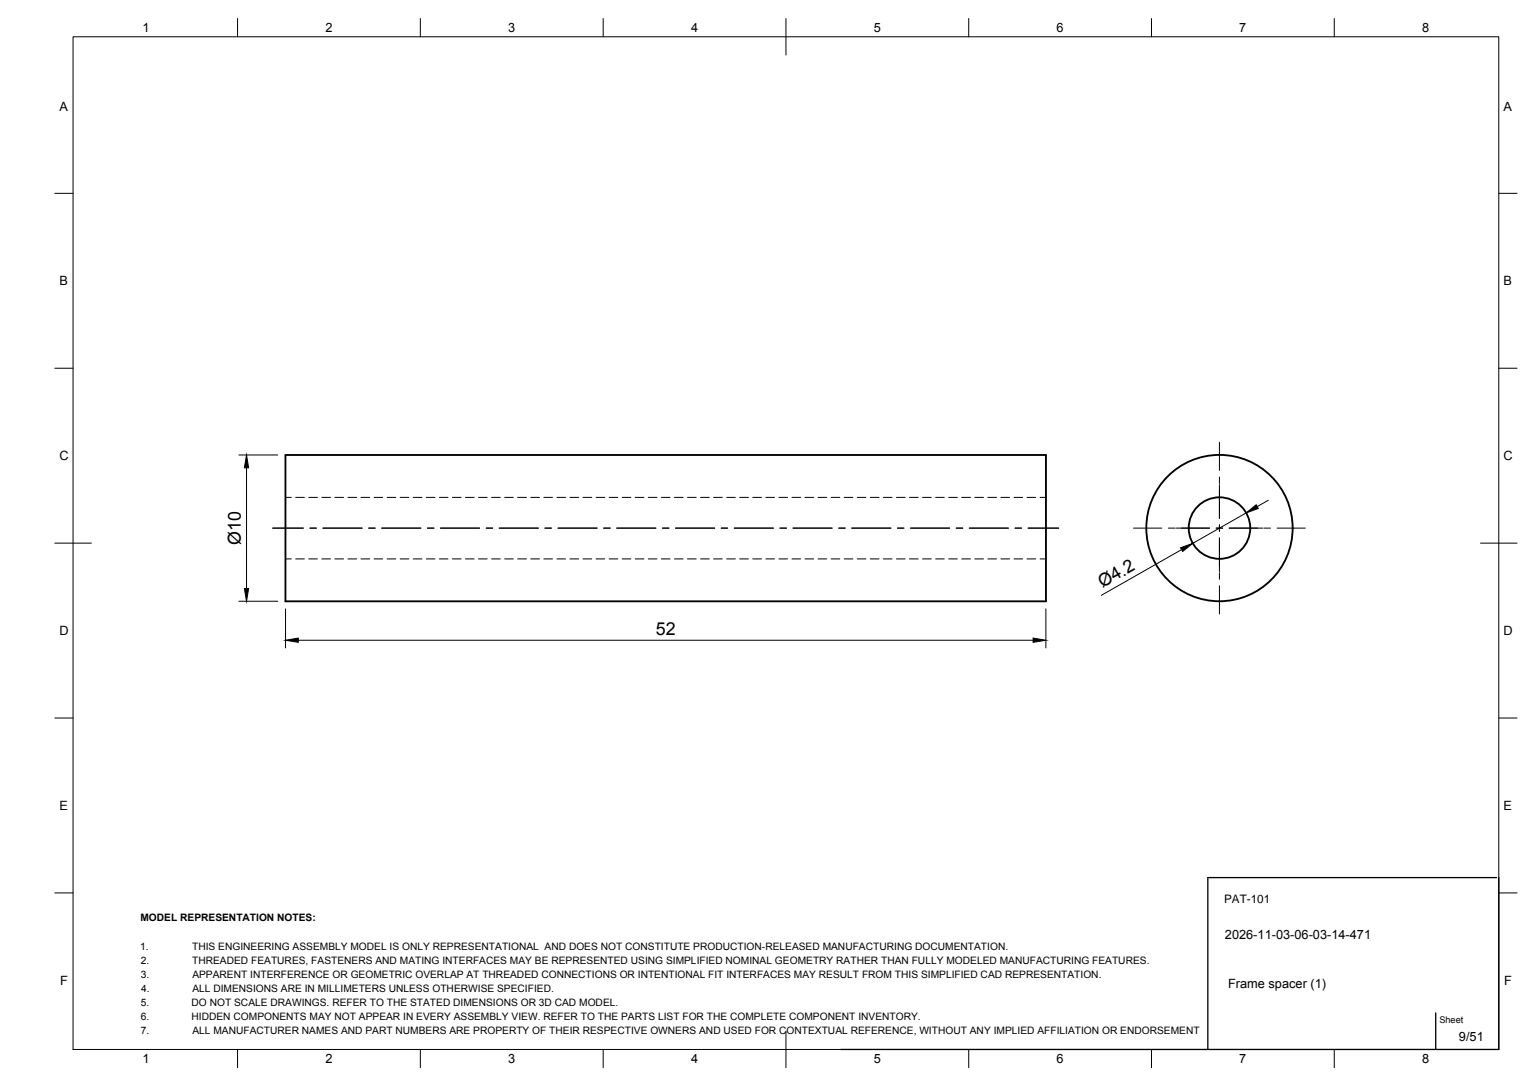
ISO-10303-21;
HEADER;
/* Generated by software containing ST-Developer
 * from STEP Tools, Inc. (www.steptools.com) 
 */

FILE_DESCRIPTION(
/* description */ ('Spur gear reduction stage 2-1 on bearing plates'),
/* implementation_level */ '2;1');

FILE_NAME(
/* name */ 'Frame spacer (1).step',
/* time_stamp */ '2026-10-28T03:22:07-07:00',
/* author */ (''),
/* organization */ (''),
/* preprocessor_version */ 'ST-DEVELOPER v20.2',
/* originating_system */ 'Autodesk Translation Framework v15.17.0.0',
/* authorisation */ '');

FILE_SCHEMA (('AUTOMOTIVE_DESIGN { 1 0 10303 214 3 1 1 }'));
ENDSEC;

DATA;
#10=MECHANICAL_DESIGN_GEOMETRIC_PRESENTATION_REPRESENTATION('',(#951),#53909);
#865=SHAPE_REPRESENTATION_RELATIONSHIP('SRR','None',#54092,#908);
#908=ADVANCED_BREP_SHAPE_REPRESENTATION('',(#1009),#53866);
#951=STYLED_ITEM('',(#54376),#1009);
#1009=MANIFOLD_SOLID_BREP('Body1',#11275);
#1134=FACE_BOUND('',#2310,.T.);
#1135=FACE_BOUND('',#2312,.T.);
#1274=PLANE('',#11993);
#1275=PLANE('',#11994);
#1585=FACE_OUTER_BOUND('',#2307,.T.);
#1586=FACE_OUTER_BOUND('',#2308,.T.);
#1587=FACE_OUTER_BOUND('',#2309,.T.);
#1588=FACE_OUTER_BOUND('',#2311,.T.);
#2307=EDGE_LOOP('',(#7700,#7701,#7702,#7703));
#2308=EDGE_LOOP('',(#7704,#7705,#7706,#7707));
#2309=EDGE_LOOP('',(#7708));
#2310=EDGE_LOOP('',(#7709));
#2311=EDGE_LOOP('',(#7710));
#2312=EDGE_LOOP('',(#7711));
#3059=LINE('',#16358,#3700);
#3060=LINE('',#16364,#3701);
#3700=VECTOR('',#13430,0.21);
#3701=VECTOR('',#13437,0.5);
#4351=CIRCLE('',#11988,0.21);
#4352=CIRCLE('',#11989,0.21);
#4353=CIRCLE('',#11991,0.5);
#4354=CIRCLE('',#11992,0.5);
#4900=VERTEX_POINT('',#16355);
#4901=VERTEX_POINT('',#16357);
#4902=VERTEX_POINT('',#16361);
#4903=VERTEX_POINT('',#16363);
#5992=EDGE_CURVE('',#4900,#4900,#4351,.T.);
#5993=EDGE_CURVE('',#4900,#4901,#3059,.T.);
#5994=EDGE_CURVE('',#4901,#4901,#4352,.T.);
#5995=EDGE_CURVE('',#4902,#4902,#4353,.T.);
#5996=EDGE_CURVE('',#4902,#4903,#3060,.T.);
#5997=EDGE_CURVE('',#4903,#4903,#4354,.T.);
#7700=ORIENTED_EDGE('',*,*,#5992,.F.);
#7701=ORIENTED_EDGE('',*,*,#5993,.T.);
#7702=ORIENTED_EDGE('',*,*,#5994,.T.);
#7703=ORIENTED_EDGE('',*,*,#5993,.F.);
#7704=ORIENTED_EDGE('',*,*,#5995,.F.);
#7705=ORIENTED_EDGE('',*,*,#5996,.T.);
#7706=ORIENTED_EDGE('',*,*,#5997,.T.);
#7707=ORIENTED_EDGE('',*,*,#5996,.F.);
#7708=ORIENTED_EDGE('',*,*,#5995,.T.);
#7709=ORIENTED_EDGE('',*,*,#5992,.T.);
#7710=ORIENTED_EDGE('',*,*,#5997,.F.);
#7711=ORIENTED_EDGE('',*,*,#5994,.F.);
#10466=CYLINDRICAL_SURFACE('',#11987,0.21);
#10467=CYLINDRICAL_SURFACE('',#11990,0.5);
#10705=ADVANCED_FACE('',(#1585),#10466,.F.);
#10706=ADVANCED_FACE('',(#1586),#10467,.T.);
#10707=ADVANCED_FACE('',(#1587,#1134),#1274,.T.);
#10708=ADVANCED_FACE('',(#1588,#1135),#1275,.F.);
#11275=CLOSED_SHELL('',(#10705,#10706,#10707,#10708));
#11986=AXIS2_PLACEMENT_3D('',#16353,#13424,#13425);
#11987=AXIS2_PLACEMENT_3D('',#16354,#13426,#13427);
#11988=AXIS2_PLACEMENT_3D('',#16356,#13428,#13429);
#11989=AXIS2_PLACEMENT_3D('',#16359,#13431,#13432);
#11990=AXIS2_PLACEMENT_3D('',#16360,#13433,#13434);
#11991=AXIS2_PLACEMENT_3D('',#16362,#13435,#13436);
#11992=AXIS2_PLACEMENT_3D('',#16365,#13438,#13439);
#11993=AXIS2_PLACEMENT_3D('',#16366,#13440,#13441);
#11994=AXIS2_PLACEMENT_3D('',#16367,#13442,#13443);
#13424=DIRECTION('axis',(0.,0.,1.));
#13425=DIRECTION('refdir',(1.,0.,0.));
#13426=DIRECTION('center_axis',(0.,1.,0.));
#13427=DIRECTION('ref_axis',(1.,0.,0.));
#13428=DIRECTION('center_axis',(0.,-1.,0.));
#13429=DIRECTION('ref_axis',(1.,0.,0.));
#13430=DIRECTION('',(0.,-1.,0.));
#13431=DIRECTION('center_axis',(0.,-1.,0.));
#13432=DIRECTION('ref_axis',(1.,0.,0.));
#13433=DIRECTION('center_axis',(0.,1.,0.));
#13434=DIRECTION('ref_axis',(1.,0.,0.));
#13435=DIRECTION('center_axis',(0.,1.,0.));
#13436=DIRECTION('ref_axis',(1.,0.,0.));
#13437=DIRECTION('',(0.,-1.,0.));
#13438=DIRECTION('center_axis',(0.,1.,0.));
#13439=DIRECTION('ref_axis',(1.,0.,0.));
#13440=DIRECTION('center_axis',(0.,1.,0.));
#13441=DIRECTION('ref_axis',(1.,0.,0.));
#13442=DIRECTION('center_axis',(0.,1.,0.));
#13443=DIRECTION('ref_axis',(1.,0.,0.));
#16353=CARTESIAN_POINT('',(0.,0.,0.));
#16354=CARTESIAN_POINT('Origin',(-2.,-2.6,9.));
#16355=CARTESIAN_POINT('',(-2.21,2.6,9.));
#16356=CARTESIAN_POINT('Origin',(-2.,2.6,9.));
#16357=CARTESIAN_POINT('',(-2.21,-2.6,9.));
#16358=CARTESIAN_POINT('',(-2.21,-2.6,9.));
#16359=CARTESIAN_POINT('Origin',(-2.,-2.6,9.));
#16360=CARTESIAN_POINT('Origin',(-2.,-2.6,9.));
#16361=CARTESIAN_POINT('',(-2.5,2.6,9.));
#16362=CARTESIAN_POINT('Origin',(-2.,2.6,9.));
#16363=CARTESIAN_POINT('',(-2.5,-2.6,9.));
#16364=CARTESIAN_POINT('',(-2.5,-2.6,9.));
#16365=CARTESIAN_POINT('Origin',(-2.,-2.6,9.));
#16366=CARTESIAN_POINT('Origin',(-2.,2.6,9.));
#16367=CARTESIAN_POINT('Origin',(-2.,-2.6,9.));
#53816=UNCERTAINTY_MEASURE_WITH_UNIT(LENGTH_MEASURE(0.001),#53910,
'DISTANCE_ACCURACY_VALUE',
'Maximum model space distance between geometric entities at asserted c
onnectivities');
#53859=UNCERTAINTY_MEASURE_WITH_UNIT(LENGTH_MEASURE(0.001),#53910,
'DISTANCE_ACCURACY_VALUE',
'Maximum model space distance between geometric entities at asserted c
onnectivities');
#53866=(
GEOMETRIC_REPRESENTATION_CONTEXT(3)
GLOBAL_UNCERTAINTY_ASSIGNED_CONTEXT((#53816))
GLOBAL_UNIT_ASSIGNED_CONTEXT((#53910,#53912,#53913))
REPRESENTATION_CONTEXT('','3D')
);
#53909=(
GEOMETRIC_REPRESENTATION_CONTEXT(3)
GLOBAL_UNCERTAINTY_ASSIGNED_CONTEXT((#53859))
GLOBAL_UNIT_ASSIGNED_CONTEXT((#53910,#53912,#53913))
REPRESENTATION_CONTEXT('','3D')
);
#53910=(
LENGTH_UNIT()
NAMED_UNIT(*)
SI_UNIT(.CENTI.,.METRE.)
);
#53912=(
NAMED_UNIT(*)
PLANE_ANGLE_UNIT()
SI_UNIT($,.RADIAN.)
);
#53913=(
NAMED_UNIT(*)
SI_UNIT($,.STERADIAN.)
SOLID_ANGLE_UNIT()
);
#53920=SHAPE_DEFINITION_REPRESENTATION(#53969,#54092);
#53969=PRODUCT_DEFINITION_SHAPE('',$,#54142);
#54092=SHAPE_REPRESENTATION('',(#11986),#53866);
#54135=PRODUCT_DEFINITION_CONTEXT('part definition',#54284,'design');
#54142=PRODUCT_DEFINITION('Frame spacer (1)','Frame spacer (1)',#54191,#54135);
#54191=PRODUCT_DEFINITION_FORMATION('',$,#54292);
#54284=APPLICATION_CONTEXT(
'Core Data for Automotive Mechanical Design Process');
#54285=PRODUCT_CONTEXT('part definition',#54284,'mechanical');
#54292=PRODUCT('Frame spacer (1)','Frame spacer (1)','Frame spacer (1)',(#54285));
#54370=COLOUR_RGB('Dark Blue',0.08,0.2,0.34);
#54371=FILL_AREA_STYLE_COLOUR('',#54370);
#54372=FILL_AREA_STYLE('',(#54371));
#54373=SURFACE_STYLE_FILL_AREA(#54372);
#54374=SURFACE_SIDE_STYLE('',(#54373));
#54375=SURFACE_STYLE_USAGE(.BOTH.,#54374);
#54376=PRESENTATION_STYLE_ASSIGNMENT((#54375));
ENDSEC;
END-ISO-10303-21;
